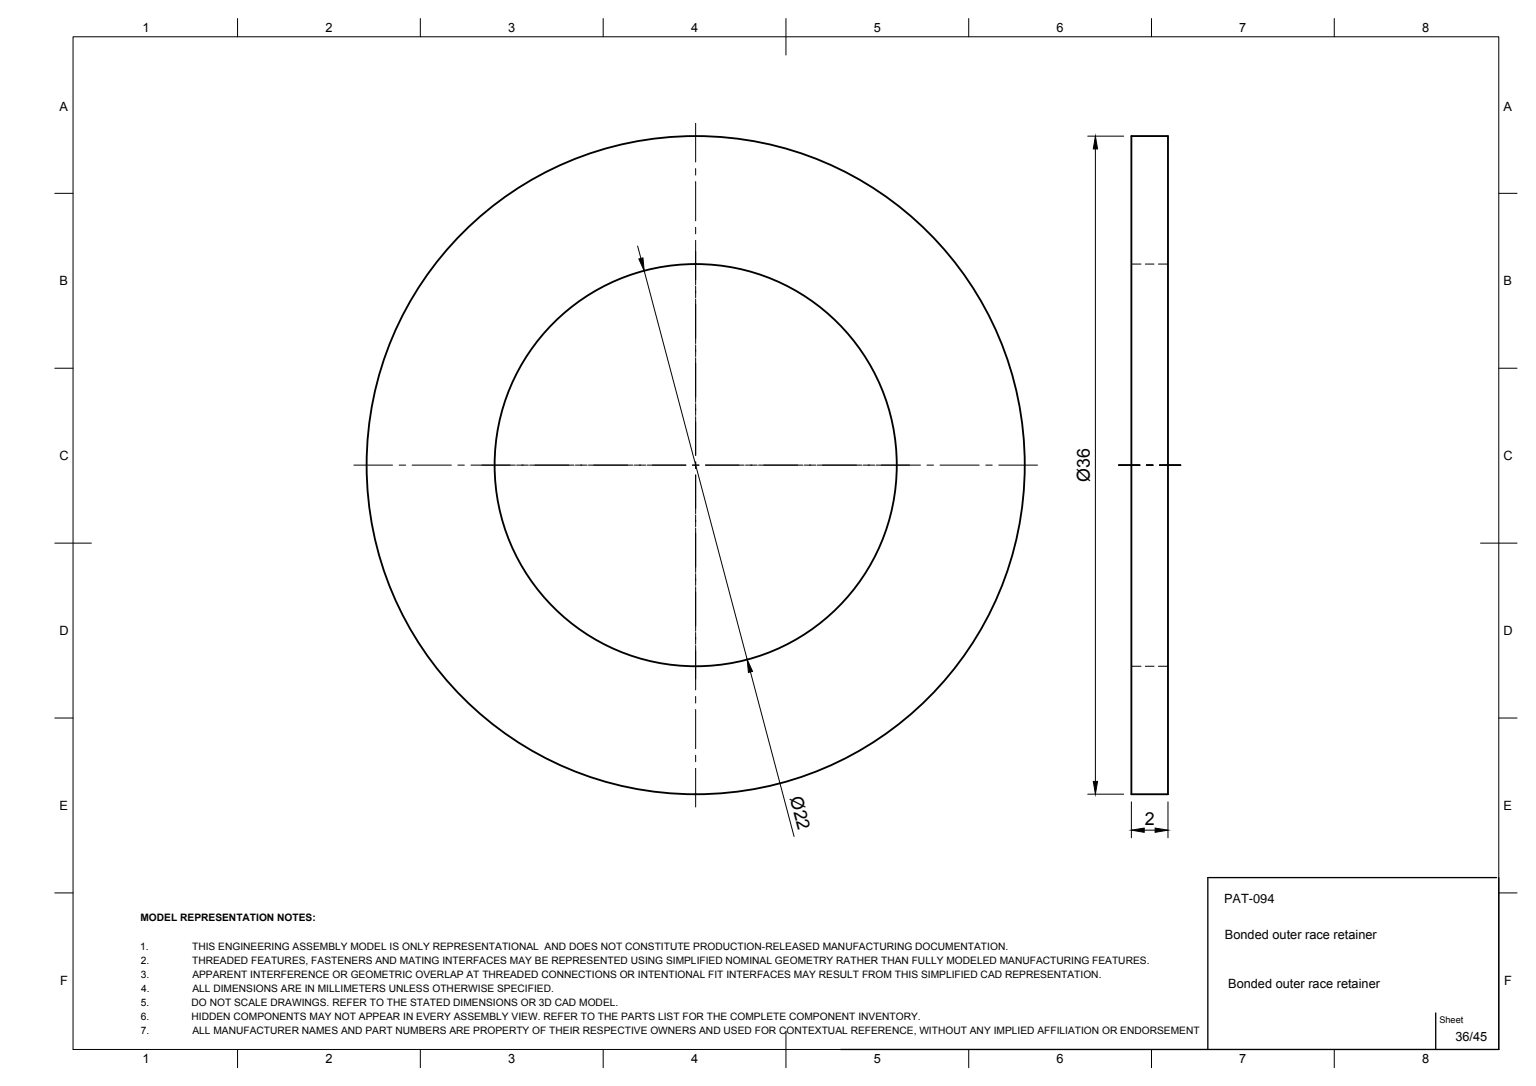
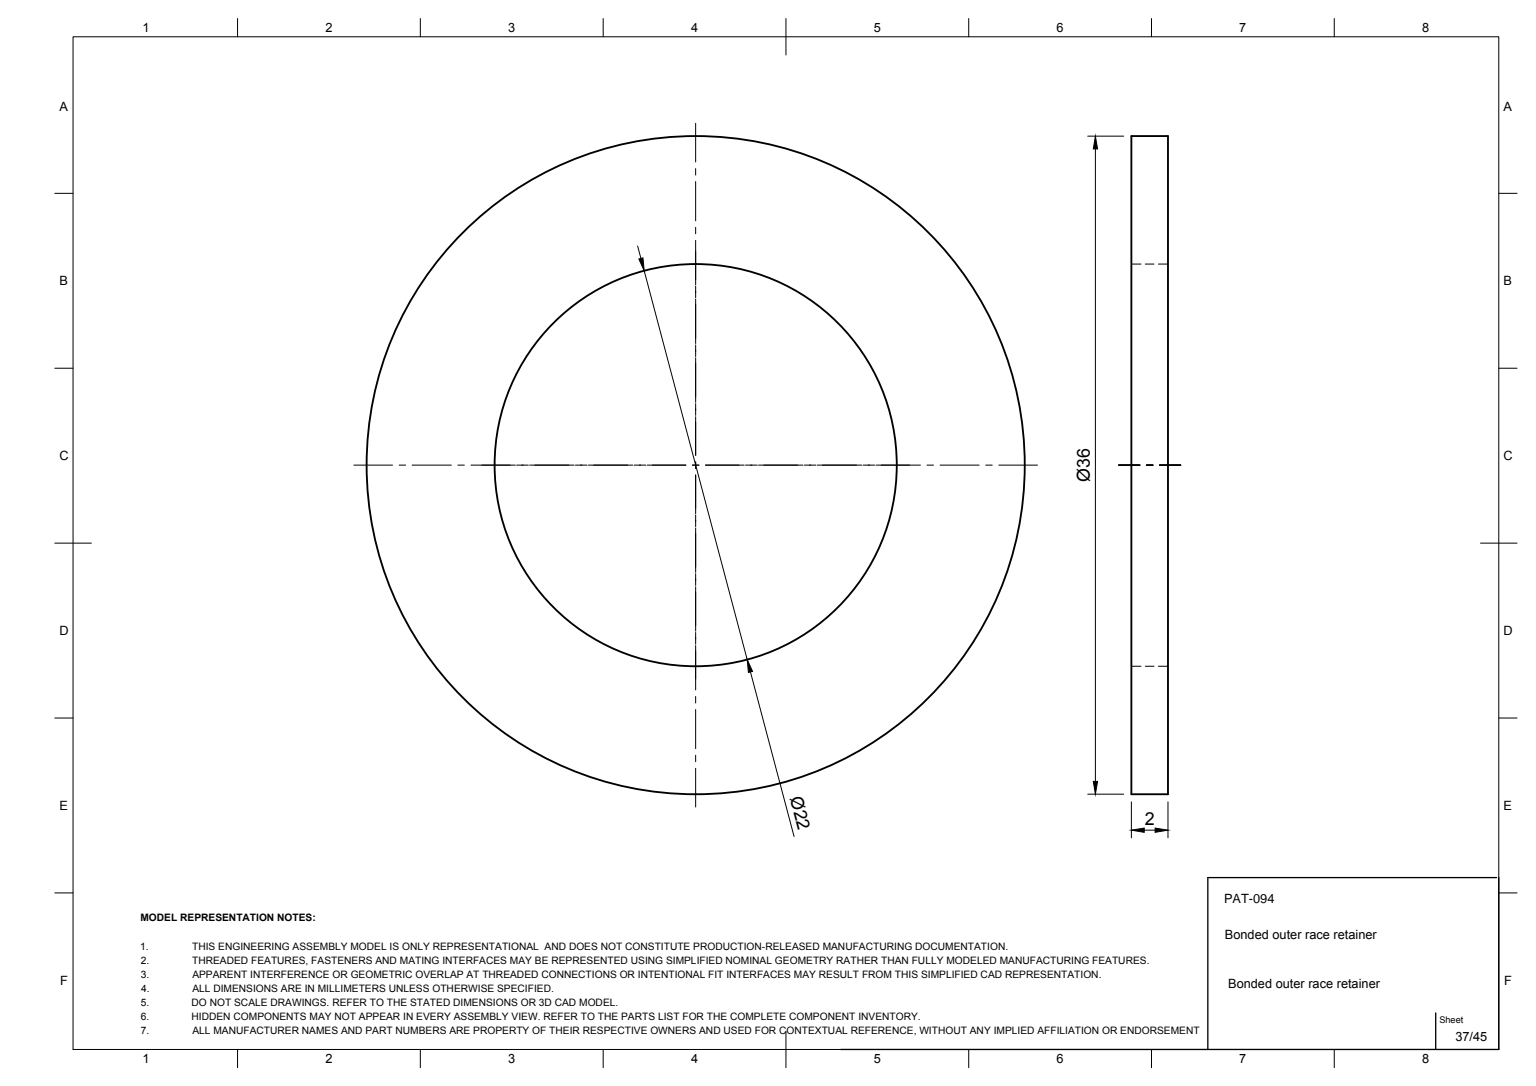
ISO-10303-21;
HEADER;
/* Generated by software containing ST-Developer
 * from STEP Tools, Inc. (www.steptools.com) 
 */

FILE_DESCRIPTION(
/* description */ ('Shaft runout checking stand'),
/* implementation_level */ '2;1');

FILE_NAME(
/* name */ 'Bonded outer race retainer.step',
/* time_stamp */ '2026-11-02T21:12:33-08:00',
/* author */ (''),
/* organization */ (''),
/* preprocessor_version */ 'ST-DEVELOPER v20.2',
/* originating_system */ 'Autodesk Translation Framework v15.17.0.0',
/* authorisation */ '');

FILE_SCHEMA (('AUTOMOTIVE_DESIGN { 1 0 10303 214 3 1 1 }'));
ENDSEC;

DATA;
#10=MECHANICAL_DESIGN_GEOMETRIC_PRESENTATION_REPRESENTATION('',(#512),#11748);
#418=SHAPE_REPRESENTATION_RELATIONSHIP('SRR','None',#11970,#461);
#461=ADVANCED_BREP_SHAPE_REPRESENTATION('',(#560),#11746);
#512=STYLED_ITEM('',(#12169),#560);
#560=MANIFOLD_SOLID_BREP('Body1',#6258);
#669=FACE_BOUND('',#1876,.T.);
#670=FACE_BOUND('',#1878,.T.);
#930=CIRCLE('',#7466,1.1);
#931=CIRCLE('',#7467,1.1);
#932=CIRCLE('',#7469,1.8);
#933=CIRCLE('',#7470,1.8);
#1034=CYLINDRICAL_SURFACE('',#7465,1.1);
#1035=CYLINDRICAL_SURFACE('',#7468,1.8);
#1398=FACE_OUTER_BOUND('',#1873,.T.);
#1399=FACE_OUTER_BOUND('',#1874,.T.);
#1400=FACE_OUTER_BOUND('',#1875,.T.);
#1401=FACE_OUTER_BOUND('',#1877,.T.);
#1873=EDGE_LOOP('',(#5580,#5581,#5582,#5583));
#1874=EDGE_LOOP('',(#5584,#5585,#5586,#5587));
#1875=EDGE_LOOP('',(#5588));
#1876=EDGE_LOOP('',(#5589));
#1877=EDGE_LOOP('',(#5590));
#1878=EDGE_LOOP('',(#5591));
#2348=LINE('',#11616,#2815);
#2349=LINE('',#11622,#2816);
#2815=VECTOR('',#9421,1.1);
#2816=VECTOR('',#9428,1.8);
#3322=VERTEX_POINT('',#11613);
#3323=VERTEX_POINT('',#11615);
#3324=VERTEX_POINT('',#11619);
#3325=VERTEX_POINT('',#11621);
#4076=EDGE_CURVE('',#3322,#3322,#930,.T.);
#4077=EDGE_CURVE('',#3322,#3323,#2348,.T.);
#4078=EDGE_CURVE('',#3323,#3323,#931,.T.);
#4079=EDGE_CURVE('',#3324,#3324,#932,.T.);
#4080=EDGE_CURVE('',#3324,#3325,#2349,.T.);
#4081=EDGE_CURVE('',#3325,#3325,#933,.T.);
#5580=ORIENTED_EDGE('',*,*,#4076,.F.);
#5581=ORIENTED_EDGE('',*,*,#4077,.T.);
#5582=ORIENTED_EDGE('',*,*,#4078,.T.);
#5583=ORIENTED_EDGE('',*,*,#4077,.F.);
#5584=ORIENTED_EDGE('',*,*,#4079,.F.);
#5585=ORIENTED_EDGE('',*,*,#4080,.T.);
#5586=ORIENTED_EDGE('',*,*,#4081,.T.);
#5587=ORIENTED_EDGE('',*,*,#4080,.F.);
#5588=ORIENTED_EDGE('',*,*,#4079,.T.);
#5589=ORIENTED_EDGE('',*,*,#4076,.T.);
#5590=ORIENTED_EDGE('',*,*,#4081,.F.);
#5591=ORIENTED_EDGE('',*,*,#4078,.F.);
#5834=PLANE('',#7471);
#5835=PLANE('',#7472);
#6198=ADVANCED_FACE('',(#1398),#1034,.F.);
#6199=ADVANCED_FACE('',(#1399),#1035,.T.);
#6200=ADVANCED_FACE('',(#1400,#669),#5834,.T.);
#6201=ADVANCED_FACE('',(#1401,#670),#5835,.F.);
#6258=CLOSED_SHELL('',(#6198,#6199,#6200,#6201));
#7464=AXIS2_PLACEMENT_3D('',#11611,#9415,#9416);
#7465=AXIS2_PLACEMENT_3D('',#11612,#9417,#9418);
#7466=AXIS2_PLACEMENT_3D('',#11614,#9419,#9420);
#7467=AXIS2_PLACEMENT_3D('',#11617,#9422,#9423);
#7468=AXIS2_PLACEMENT_3D('',#11618,#9424,#9425);
#7469=AXIS2_PLACEMENT_3D('',#11620,#9426,#9427);
#7470=AXIS2_PLACEMENT_3D('',#11623,#9429,#9430);
#7471=AXIS2_PLACEMENT_3D('',#11624,#9431,#9432);
#7472=AXIS2_PLACEMENT_3D('',#11625,#9433,#9434);
#9415=DIRECTION('axis',(0.,0.,1.));
#9416=DIRECTION('refdir',(1.,0.,0.));
#9417=DIRECTION('center_axis',(0.,1.,0.));
#9418=DIRECTION('ref_axis',(1.,0.,0.));
#9419=DIRECTION('center_axis',(0.,-1.,0.));
#9420=DIRECTION('ref_axis',(1.,0.,0.));
#9421=DIRECTION('',(0.,-1.,0.));
#9422=DIRECTION('center_axis',(0.,-1.,0.));
#9423=DIRECTION('ref_axis',(1.,0.,0.));
#9424=DIRECTION('center_axis',(0.,1.,0.));
#9425=DIRECTION('ref_axis',(1.,0.,0.));
#9426=DIRECTION('center_axis',(0.,1.,0.));
#9427=DIRECTION('ref_axis',(1.,0.,0.));
#9428=DIRECTION('',(0.,-1.,0.));
#9429=DIRECTION('center_axis',(0.,1.,0.));
#9430=DIRECTION('ref_axis',(1.,0.,0.));
#9431=DIRECTION('center_axis',(0.,1.,0.));
#9432=DIRECTION('ref_axis',(1.,0.,0.));
#9433=DIRECTION('center_axis',(0.,1.,0.));
#9434=DIRECTION('ref_axis',(1.,0.,0.));
#11611=CARTESIAN_POINT('',(0.,0.,0.));
#11612=CARTESIAN_POINT('Origin',(-2.,-10.65,5.));
#11613=CARTESIAN_POINT('',(-3.1,-10.45,5.));
#11614=CARTESIAN_POINT('Origin',(-2.,-10.45,5.));
#11615=CARTESIAN_POINT('',(-3.1,-10.65,5.));
#11616=CARTESIAN_POINT('',(-3.1,-10.65,5.));
#11617=CARTESIAN_POINT('Origin',(-2.,-10.65,5.));
#11618=CARTESIAN_POINT('Origin',(-2.,-10.65,5.));
#11619=CARTESIAN_POINT('',(-3.8,-10.45,5.));
#11620=CARTESIAN_POINT('Origin',(-2.,-10.45,5.));
#11621=CARTESIAN_POINT('',(-3.8,-10.65,5.));
#11622=CARTESIAN_POINT('',(-3.8,-10.65,5.));
#11623=CARTESIAN_POINT('Origin',(-2.,-10.65,5.));
#11624=CARTESIAN_POINT('Origin',(-2.,-10.45,5.));
#11625=CARTESIAN_POINT('Origin',(-2.,-10.65,5.));
#11697=UNCERTAINTY_MEASURE_WITH_UNIT(LENGTH_MEASURE(0.001),#11749,
'DISTANCE_ACCURACY_VALUE',
'Maximum model space distance between geometric entities at asserted c
onnectivities');
#11699=UNCERTAINTY_MEASURE_WITH_UNIT(LENGTH_MEASURE(0.001),#11749,
'DISTANCE_ACCURACY_VALUE',
'Maximum model space distance between geometric entities at asserted c
onnectivities');
#11746=(
GEOMETRIC_REPRESENTATION_CONTEXT(3)
GLOBAL_UNCERTAINTY_ASSIGNED_CONTEXT((#11697))
GLOBAL_UNIT_ASSIGNED_CONTEXT((#11749,#11751,#11752))
REPRESENTATION_CONTEXT('','3D')
);
#11748=(
GEOMETRIC_REPRESENTATION_CONTEXT(3)
GLOBAL_UNCERTAINTY_ASSIGNED_CONTEXT((#11699))
GLOBAL_UNIT_ASSIGNED_CONTEXT((#11749,#11751,#11752))
REPRESENTATION_CONTEXT('','3D')
);
#11749=(
LENGTH_UNIT()
NAMED_UNIT(*)
SI_UNIT(.CENTI.,.METRE.)
);
#11751=(
NAMED_UNIT(*)
PLANE_ANGLE_UNIT()
SI_UNIT($,.RADIAN.)
);
#11752=(
NAMED_UNIT(*)
SI_UNIT($,.STERADIAN.)
SOLID_ANGLE_UNIT()
);
#11799=SHAPE_DEFINITION_REPRESENTATION(#11912,#11970);
#11912=PRODUCT_DEFINITION_SHAPE('',$,#12019);
#11970=SHAPE_REPRESENTATION('',(#7464),#11746);
#11972=PRODUCT_DEFINITION_CONTEXT('part definition',#12118,'design');
#12019=PRODUCT_DEFINITION('Bonded outer race retainer',
'Bonded outer race retainer',#12067,#11972);
#12067=PRODUCT_DEFINITION_FORMATION('',$,#12166);
#12118=APPLICATION_CONTEXT(
'Core Data for Automotive Mechanical Design Process');
#12119=PRODUCT_CONTEXT('part definition',#12118,'mechanical');
#12166=PRODUCT('Bonded outer race retainer',
'Bonded outer race retainer','Bonded outer race retainer',(#12119));
#12169=PRESENTATION_STYLE_ASSIGNMENT((#12174));
#12174=SURFACE_STYLE_USAGE(.BOTH.,#12179);
#12179=SURFACE_SIDE_STYLE('',(#12184));
#12184=SURFACE_STYLE_FILL_AREA(#12189);
#12189=FILL_AREA_STYLE('CAD Library Painted - Engineering blue',(#12194));
#12194=FILL_AREA_STYLE_COLOUR('CAD Library Painted - Engineering blue',
#12199);
#12199=COLOUR_RGB('CAD Library Painted - Engineering blue',0.12156862745098,
0.356862745098039,0.6);
ENDSEC;
END-ISO-10303-21;
